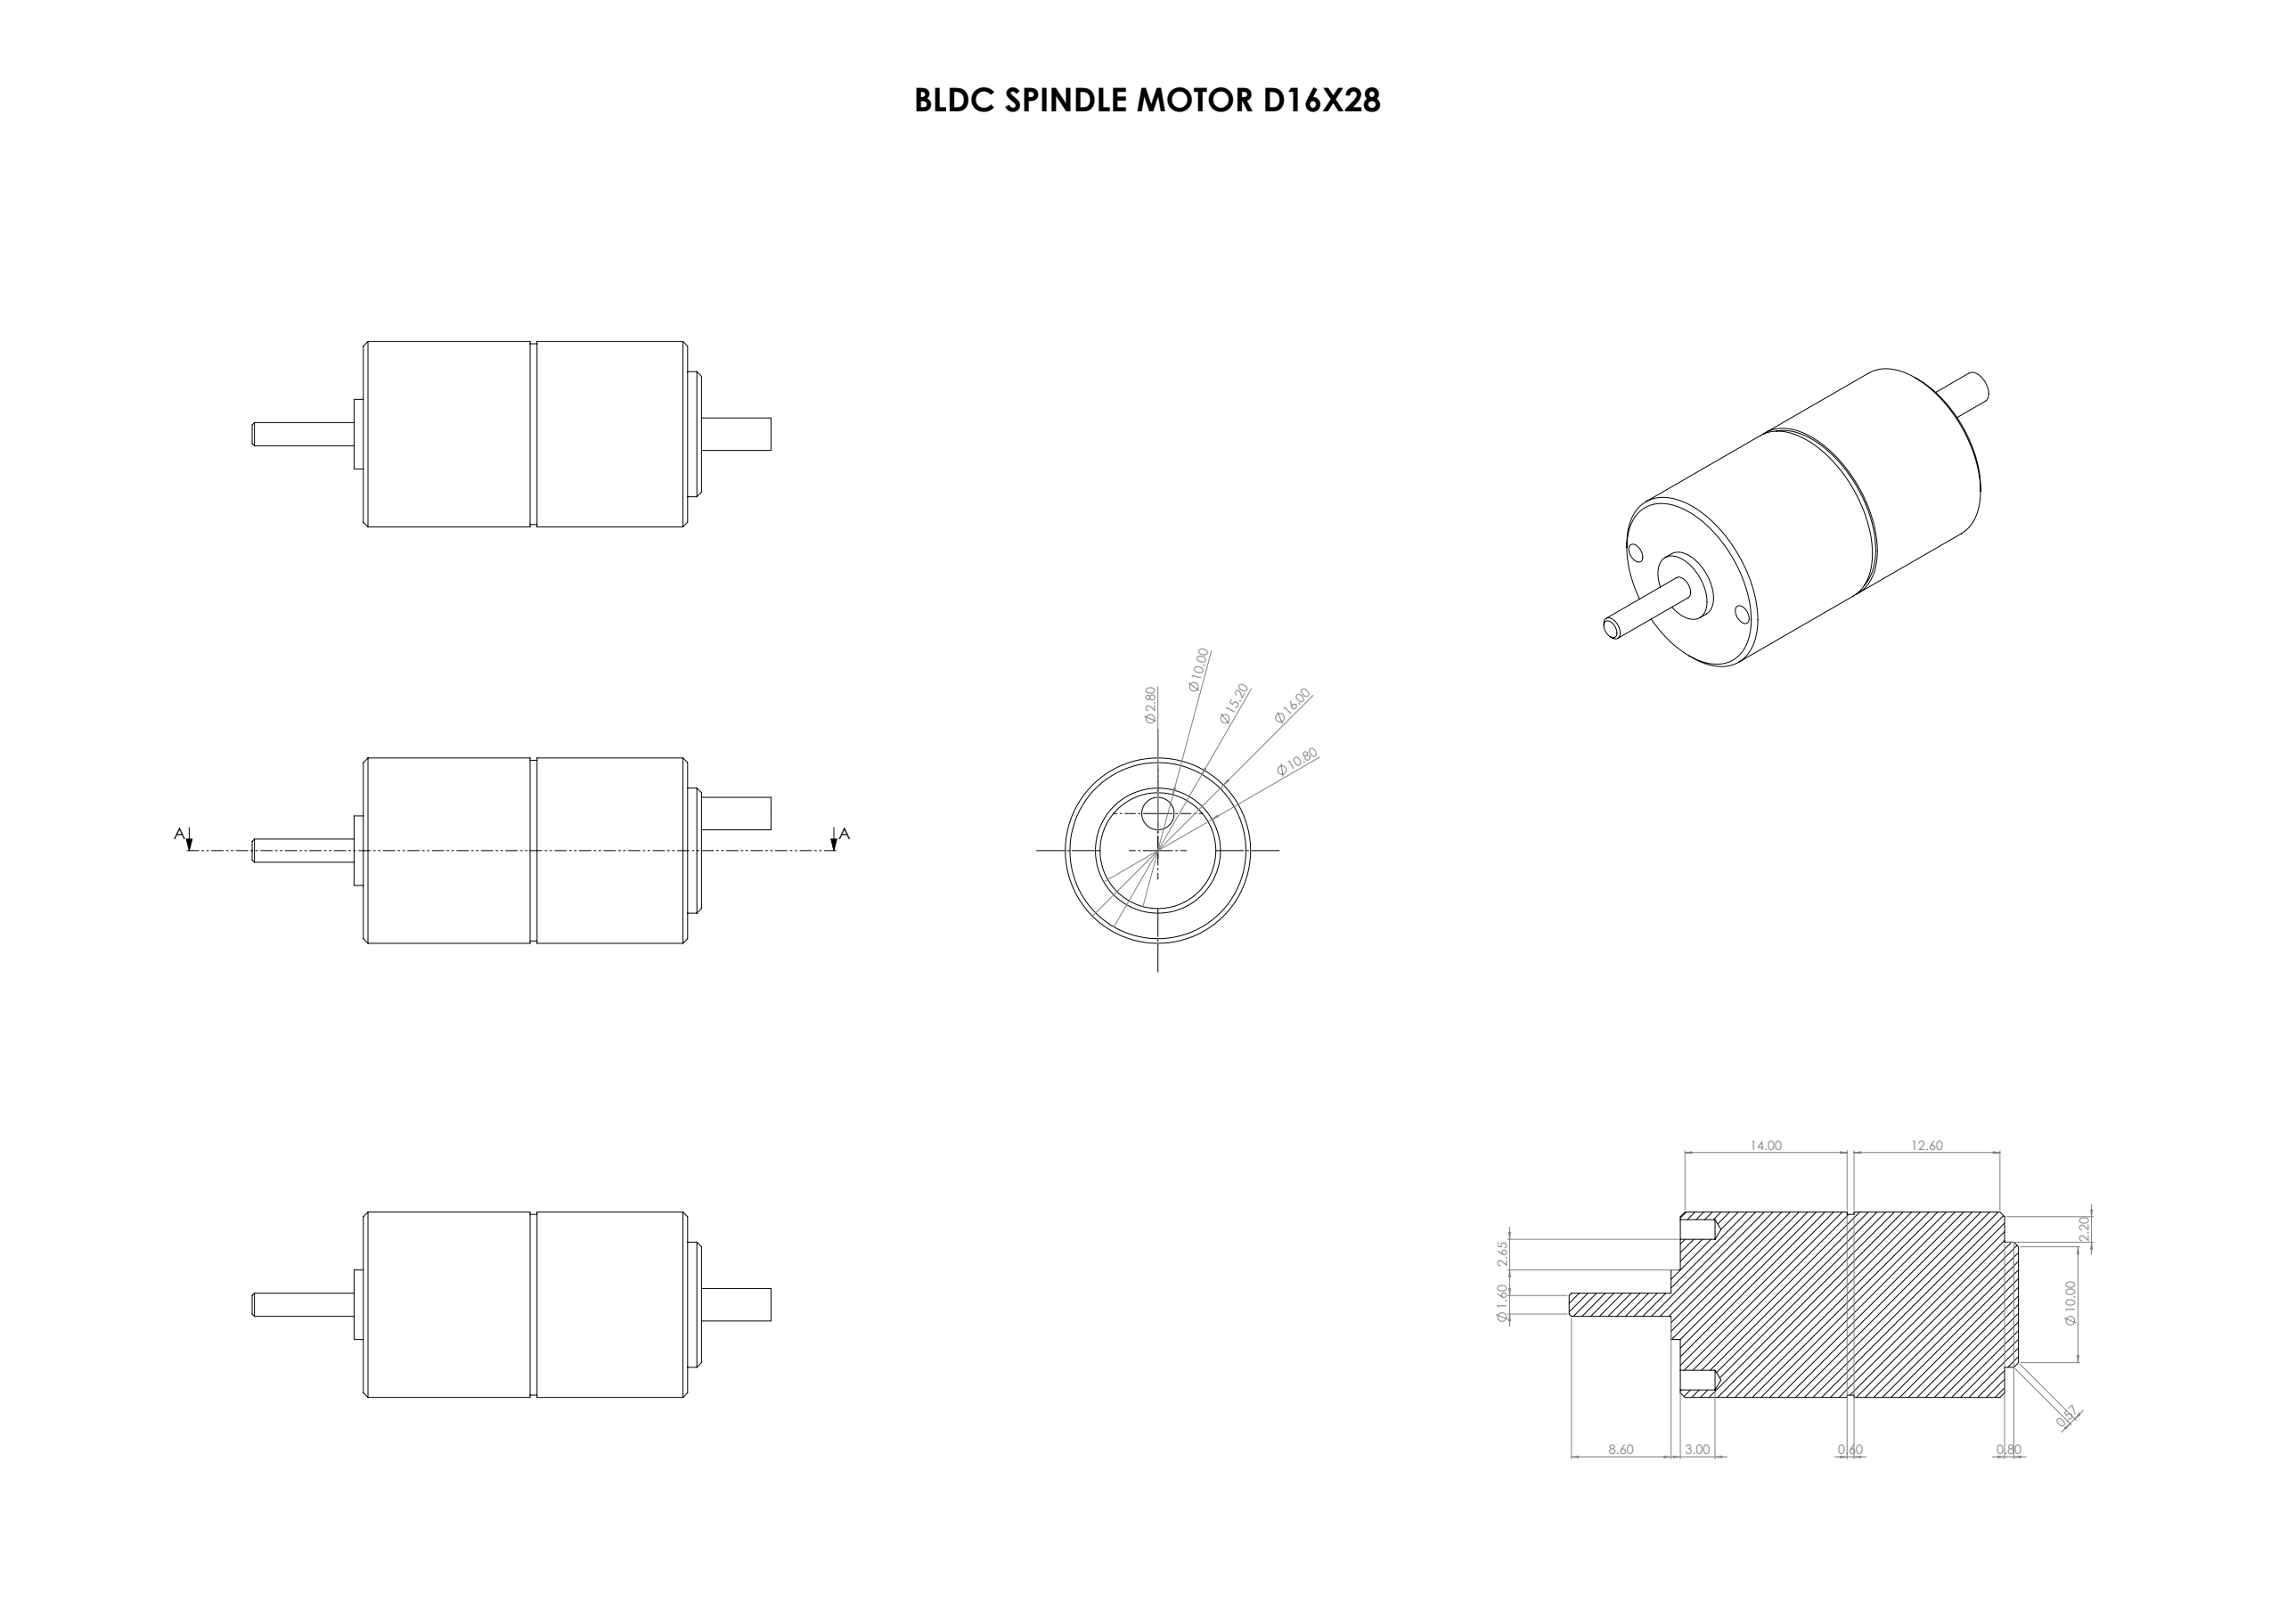
ISO-10303-21;
HEADER;
/* Generated by software containing ST-Developer
 * from STEP Tools, Inc. (www.steptools.com) 
 */

FILE_DESCRIPTION(
/* description */ (''),
/* implementation_level */ '2;1');

FILE_NAME(
/* name */ '07_BLDC_Spindle_Motor_D16x28.step',
/* time_stamp */ '2026-10-19T23:00:43-07:00',
/* author */ (''),
/* organization */ (''),
/* preprocessor_version */ 'ST-DEVELOPER v20.2',
/* originating_system */ 'Autodesk Translation Framework v15.15.0.0',
/* authorisation */ '');

FILE_SCHEMA (('AUTOMOTIVE_DESIGN { 1 0 10303 214 3 1 1 }'));
ENDSEC;

DATA;
#10=MECHANICAL_DESIGN_GEOMETRIC_PRESENTATION_REPRESENTATION('',(#1002),#55002);
#962=SHAPE_REPRESENTATION_RELATIONSHIP('SRR','None',#55110,#982);
#982=ADVANCED_BREP_SHAPE_REPRESENTATION('',(#1022),#54988);
#1002=STYLED_ITEM('',(#55372),#1022);
#1022=MANIFOLD_SOLID_BREP('BLDC Motor',#24535);
#1189=FACE_BOUND('',#4421,.T.);
#1190=FACE_BOUND('',#4426,.T.);
#1191=FACE_BOUND('',#4428,.T.);
#1192=FACE_BOUND('',#4431,.T.);
#1193=FACE_BOUND('',#4436,.T.);
#1194=FACE_BOUND('',#4437,.T.);
#1195=FACE_BOUND('',#4438,.T.);
#1196=FACE_BOUND('',#4441,.T.);
#1425=PLANE('',#25811);
#1426=PLANE('',#25812);
#1427=PLANE('',#25821);
#1428=PLANE('',#25823);
#1429=PLANE('',#25827);
#1430=PLANE('',#25834);
#1431=PLANE('',#25838);
#1432=PLANE('',#25844);
#2139=CYLINDRICAL_SURFACE('',#25802,0.085);
#2140=CYLINDRICAL_SURFACE('',#25806,0.085);
#2141=CYLINDRICAL_SURFACE('',#25808,0.14);
#2142=CYLINDRICAL_SURFACE('',#25816,0.54);
#2143=CYLINDRICAL_SURFACE('',#25818,0.78);
#2144=CYLINDRICAL_SURFACE('',#25825,0.8);
#2145=CYLINDRICAL_SURFACE('',#25831,0.8);
#2146=CYLINDRICAL_SURFACE('',#25836,0.3);
#2147=CYLINDRICAL_SURFACE('',#25840,0.1);
#2897=FACE_OUTER_BOUND('',#4414,.T.);
#2898=FACE_OUTER_BOUND('',#4415,.T.);
#2899=FACE_OUTER_BOUND('',#4416,.T.);
#2900=FACE_OUTER_BOUND('',#4417,.T.);
#2901=FACE_OUTER_BOUND('',#4418,.T.);
#2902=FACE_OUTER_BOUND('',#4419,.T.);
#2903=FACE_OUTER_BOUND('',#4420,.T.);
#2904=FACE_OUTER_BOUND('',#4422,.T.);
#2905=FACE_OUTER_BOUND('',#4423,.T.);
#2906=FACE_OUTER_BOUND('',#4424,.T.);
#2907=FACE_OUTER_BOUND('',#4425,.T.);
#2908=FACE_OUTER_BOUND('',#4427,.T.);
#2909=FACE_OUTER_BOUND('',#4429,.T.);
#2910=FACE_OUTER_BOUND('',#4430,.T.);
#2911=FACE_OUTER_BOUND('',#4432,.T.);
#2912=FACE_OUTER_BOUND('',#4433,.T.);
#2913=FACE_OUTER_BOUND('',#4434,.T.);
#2914=FACE_OUTER_BOUND('',#4435,.T.);
#2915=FACE_OUTER_BOUND('',#4439,.T.);
#2916=FACE_OUTER_BOUND('',#4440,.T.);
#2917=FACE_OUTER_BOUND('',#4442,.T.);
#2918=FACE_OUTER_BOUND('',#4443,.T.);
#2919=FACE_OUTER_BOUND('',#4444,.T.);
#4414=EDGE_LOOP('',(#18100,#18101,#18102));
#4415=EDGE_LOOP('',(#18103,#18104,#18105,#18106));
#4416=EDGE_LOOP('',(#18107,#18108,#18109));
#4417=EDGE_LOOP('',(#18110,#18111,#18112,#18113));
#4418=EDGE_LOOP('',(#18114,#18115,#18116,#18117));
#4419=EDGE_LOOP('',(#18118));
#4420=EDGE_LOOP('',(#18119));
#4421=EDGE_LOOP('',(#18120));
#4422=EDGE_LOOP('',(#18121,#18122,#18123,#18124));
#4423=EDGE_LOOP('',(#18125,#18126,#18127,#18128));
#4424=EDGE_LOOP('',(#18129,#18130,#18131,#18132));
#4425=EDGE_LOOP('',(#18133));
#4426=EDGE_LOOP('',(#18134));
#4427=EDGE_LOOP('',(#18135));
#4428=EDGE_LOOP('',(#18136));
#4429=EDGE_LOOP('',(#18137,#18138,#18139,#18140));
#4430=EDGE_LOOP('',(#18141));
#4431=EDGE_LOOP('',(#18142));
#4432=EDGE_LOOP('',(#18143,#18144,#18145,#18146));
#4433=EDGE_LOOP('',(#18147,#18148,#18149,#18150));
#4434=EDGE_LOOP('',(#18151,#18152,#18153,#18154));
#4435=EDGE_LOOP('',(#18155));
#4436=EDGE_LOOP('',(#18156));
#4437=EDGE_LOOP('',(#18157));
#4438=EDGE_LOOP('',(#18158));
#4439=EDGE_LOOP('',(#18159,#18160,#18161,#18162));
#4440=EDGE_LOOP('',(#18163));
#4441=EDGE_LOOP('',(#18164));
#4442=EDGE_LOOP('',(#18165,#18166,#18167,#18168));
#4443=EDGE_LOOP('',(#18169,#18170,#18171,#18172));
#4444=EDGE_LOOP('',(#18173));
#5948=LINE('',#36207,#7769);
#5949=LINE('',#36211,#7770);
#5950=LINE('',#36216,#7771);
#5951=LINE('',#36220,#7772);
#5952=LINE('',#36226,#7773);
#5953=LINE('',#36235,#7774);
#5954=LINE('',#36239,#7775);
#5955=LINE('',#36244,#7776);
#5956=LINE('',#36255,#7777);
#5957=LINE('',#36262,#7778);
#5958=LINE('',#36264,#7779);
#5959=LINE('',#36268,#7780);
#5960=LINE('',#36275,#7781);
#5961=LINE('',#36282,#7782);
#5962=LINE('',#36286,#7783);
#7769=VECTOR('',#29826,0.0425);
#7770=VECTOR('',#29831,0.085);
#7771=VECTOR('',#29836,0.0425);
#7772=VECTOR('',#29841,0.085);
#7773=VECTOR('',#29848,0.14);
#7774=VECTOR('',#29861,0.52);
#7775=VECTOR('',#29866,0.54);
#7776=VECTOR('',#29871,0.78);
#7777=VECTOR('',#29886,0.8);
#7778=VECTOR('',#29895,0.78);
#7779=VECTOR('',#29898,0.8);
#7780=VECTOR('',#29903,0.78);
#7781=VECTOR('',#29912,0.3);
#7782=VECTOR('',#29921,0.1);
#7783=VECTOR('',#29926,0.09);
#9559=CIRCLE('',#25801,0.085);
#9560=CIRCLE('',#25803,0.085);
#9561=CIRCLE('',#25805,0.085);
#9562=CIRCLE('',#25807,0.085);
#9563=CIRCLE('',#25809,0.14);
#9564=CIRCLE('',#25810,0.14);
#9565=CIRCLE('',#25813,0.5);
#9566=CIRCLE('',#25815,0.54);
#9567=CIRCLE('',#25817,0.54);
#9568=CIRCLE('',#25819,0.78);
#9569=CIRCLE('',#25820,0.78);
#9570=CIRCLE('',#25822,0.8);
#9571=CIRCLE('',#25824,0.8);
#9572=CIRCLE('',#25826,0.8);
#9573=CIRCLE('',#25828,0.76);
#9574=CIRCLE('',#25830,0.8);
#9575=CIRCLE('',#25833,0.76);
#9576=CIRCLE('',#25835,0.3);
#9577=CIRCLE('',#25837,0.3);
#9578=CIRCLE('',#25839,0.1);
#9579=CIRCLE('',#25841,0.1);
#9580=CIRCLE('',#25843,0.08);
#10743=VERTEX_POINT('',#36205);
#10744=VERTEX_POINT('',#36206);
#10745=VERTEX_POINT('',#36210);
#10746=VERTEX_POINT('',#36214);
#10747=VERTEX_POINT('',#36215);
#10748=VERTEX_POINT('',#36219);
#10749=VERTEX_POINT('',#36223);
#10750=VERTEX_POINT('',#36225);
#10751=VERTEX_POINT('',#36230);
#10752=VERTEX_POINT('',#36233);
#10753=VERTEX_POINT('',#36237);
#10754=VERTEX_POINT('',#36241);
#10755=VERTEX_POINT('',#36243);
#10756=VERTEX_POINT('',#36247);
#10757=VERTEX_POINT('',#36250);
#10758=VERTEX_POINT('',#36253);
#10759=VERTEX_POINT('',#36257);
#10760=VERTEX_POINT('',#36260);
#10761=VERTEX_POINT('',#36266);
#10762=VERTEX_POINT('',#36270);
#10763=VERTEX_POINT('',#36273);
#10764=VERTEX_POINT('',#36277);
#10765=VERTEX_POINT('',#36280);
#10766=VERTEX_POINT('',#36284);
#13458=EDGE_CURVE('',#10743,#10744,#5948,.T.);
#13459=EDGE_CURVE('',#10744,#10744,#9559,.T.);
#13460=EDGE_CURVE('',#10744,#10745,#5949,.T.);
#13461=EDGE_CURVE('',#10745,#10745,#9560,.T.);
#13462=EDGE_CURVE('',#10746,#10747,#5950,.T.);
#13463=EDGE_CURVE('',#10747,#10747,#9561,.T.);
#13464=EDGE_CURVE('',#10747,#10748,#5951,.T.);
#13465=EDGE_CURVE('',#10748,#10748,#9562,.T.);
#13466=EDGE_CURVE('',#10749,#10749,#9563,.T.);
#13467=EDGE_CURVE('',#10749,#10750,#5952,.T.);
#13468=EDGE_CURVE('',#10750,#10750,#9564,.T.);
#13469=EDGE_CURVE('',#10751,#10751,#9565,.T.);
#13470=EDGE_CURVE('',#10752,#10752,#9566,.T.);
#13471=EDGE_CURVE('',#10752,#10751,#5953,.T.);
#13472=EDGE_CURVE('',#10753,#10753,#9567,.T.);
#13473=EDGE_CURVE('',#10753,#10752,#5954,.T.);
#13474=EDGE_CURVE('',#10754,#10754,#9568,.T.);
#13475=EDGE_CURVE('',#10754,#10755,#5955,.T.);
#13476=EDGE_CURVE('',#10755,#10755,#9569,.T.);
#13477=EDGE_CURVE('',#10756,#10756,#9570,.T.);
#13478=EDGE_CURVE('',#10757,#10757,#9571,.T.);
#13479=EDGE_CURVE('',#10758,#10758,#9572,.T.);
#13480=EDGE_CURVE('',#10758,#10757,#5956,.T.);
#13481=EDGE_CURVE('',#10759,#10759,#9573,.T.);
#13482=EDGE_CURVE('',#10760,#10760,#9574,.T.);
#13483=EDGE_CURVE('',#10760,#10759,#5957,.T.);
#13484=EDGE_CURVE('',#10756,#10760,#5958,.T.);
#13485=EDGE_CURVE('',#10761,#10761,#9575,.T.);
#13486=EDGE_CURVE('',#10761,#10758,#5959,.T.);
#13487=EDGE_CURVE('',#10762,#10762,#9576,.T.);
#13488=EDGE_CURVE('',#10763,#10763,#9577,.T.);
#13489=EDGE_CURVE('',#10763,#10762,#5960,.T.);
#13490=EDGE_CURVE('',#10764,#10764,#9578,.T.);
#13491=EDGE_CURVE('',#10765,#10765,#9579,.T.);
#13492=EDGE_CURVE('',#10765,#10764,#5961,.T.);
#13493=EDGE_CURVE('',#10766,#10766,#9580,.T.);
#13494=EDGE_CURVE('',#10766,#10765,#5962,.T.);
#18100=ORIENTED_EDGE('',*,*,#13458,.T.);
#18101=ORIENTED_EDGE('',*,*,#13459,.T.);
#18102=ORIENTED_EDGE('',*,*,#13458,.F.);
#18103=ORIENTED_EDGE('',*,*,#13459,.F.);
#18104=ORIENTED_EDGE('',*,*,#13460,.T.);
#18105=ORIENTED_EDGE('',*,*,#13461,.F.);
#18106=ORIENTED_EDGE('',*,*,#13460,.F.);
#18107=ORIENTED_EDGE('',*,*,#13462,.T.);
#18108=ORIENTED_EDGE('',*,*,#13463,.T.);
#18109=ORIENTED_EDGE('',*,*,#13462,.F.);
#18110=ORIENTED_EDGE('',*,*,#13463,.F.);
#18111=ORIENTED_EDGE('',*,*,#13464,.T.);
#18112=ORIENTED_EDGE('',*,*,#13465,.F.);
#18113=ORIENTED_EDGE('',*,*,#13464,.F.);
#18114=ORIENTED_EDGE('',*,*,#13466,.F.);
#18115=ORIENTED_EDGE('',*,*,#13467,.T.);
#18116=ORIENTED_EDGE('',*,*,#13468,.F.);
#18117=ORIENTED_EDGE('',*,*,#13467,.F.);
#18118=ORIENTED_EDGE('',*,*,#13466,.T.);
#18119=ORIENTED_EDGE('',*,*,#13469,.F.);
#18120=ORIENTED_EDGE('',*,*,#13468,.T.);
#18121=ORIENTED_EDGE('',*,*,#13470,.F.);
#18122=ORIENTED_EDGE('',*,*,#13471,.T.);
#18123=ORIENTED_EDGE('',*,*,#13469,.T.);
#18124=ORIENTED_EDGE('',*,*,#13471,.F.);
#18125=ORIENTED_EDGE('',*,*,#13472,.F.);
#18126=ORIENTED_EDGE('',*,*,#13473,.T.);
#18127=ORIENTED_EDGE('',*,*,#13470,.T.);
#18128=ORIENTED_EDGE('',*,*,#13473,.F.);
#18129=ORIENTED_EDGE('',*,*,#13474,.T.);
#18130=ORIENTED_EDGE('',*,*,#13475,.T.);
#18131=ORIENTED_EDGE('',*,*,#13476,.F.);
#18132=ORIENTED_EDGE('',*,*,#13475,.F.);
#18133=ORIENTED_EDGE('',*,*,#13477,.F.);
#18134=ORIENTED_EDGE('',*,*,#13474,.F.);
#18135=ORIENTED_EDGE('',*,*,#13478,.F.);
#18136=ORIENTED_EDGE('',*,*,#13476,.T.);
#18137=ORIENTED_EDGE('',*,*,#13479,.F.);
#18138=ORIENTED_EDGE('',*,*,#13480,.T.);
#18139=ORIENTED_EDGE('',*,*,#13478,.T.);
#18140=ORIENTED_EDGE('',*,*,#13480,.F.);
#18141=ORIENTED_EDGE('',*,*,#13481,.F.);
#18142=ORIENTED_EDGE('',*,*,#13472,.T.);
#18143=ORIENTED_EDGE('',*,*,#13482,.F.);
#18144=ORIENTED_EDGE('',*,*,#13483,.T.);
#18145=ORIENTED_EDGE('',*,*,#13481,.T.);
#18146=ORIENTED_EDGE('',*,*,#13483,.F.);
#18147=ORIENTED_EDGE('',*,*,#13477,.T.);
#18148=ORIENTED_EDGE('',*,*,#13484,.T.);
#18149=ORIENTED_EDGE('',*,*,#13482,.T.);
#18150=ORIENTED_EDGE('',*,*,#13484,.F.);
#18151=ORIENTED_EDGE('',*,*,#13485,.F.);
#18152=ORIENTED_EDGE('',*,*,#13486,.T.);
#18153=ORIENTED_EDGE('',*,*,#13479,.T.);
#18154=ORIENTED_EDGE('',*,*,#13486,.F.);
#18155=ORIENTED_EDGE('',*,*,#13485,.T.);
#18156=ORIENTED_EDGE('',*,*,#13461,.T.);
#18157=ORIENTED_EDGE('',*,*,#13465,.T.);
#18158=ORIENTED_EDGE('',*,*,#13487,.F.);
#18159=ORIENTED_EDGE('',*,*,#13488,.F.);
#18160=ORIENTED_EDGE('',*,*,#13489,.T.);
#18161=ORIENTED_EDGE('',*,*,#13487,.T.);
#18162=ORIENTED_EDGE('',*,*,#13489,.F.);
#18163=ORIENTED_EDGE('',*,*,#13488,.T.);
#18164=ORIENTED_EDGE('',*,*,#13490,.F.);
#18165=ORIENTED_EDGE('',*,*,#13491,.F.);
#18166=ORIENTED_EDGE('',*,*,#13492,.T.);
#18167=ORIENTED_EDGE('',*,*,#13490,.T.);
#18168=ORIENTED_EDGE('',*,*,#13492,.F.);
#18169=ORIENTED_EDGE('',*,*,#13493,.F.);
#18170=ORIENTED_EDGE('',*,*,#13494,.T.);
#18171=ORIENTED_EDGE('',*,*,#13491,.T.);
#18172=ORIENTED_EDGE('',*,*,#13494,.F.);
#18173=ORIENTED_EDGE('',*,*,#13493,.T.);
#23103=CONICAL_SURFACE('',#25800,0.0425,1.02974425867665);
#23104=CONICAL_SURFACE('',#25804,0.0425,1.02974425867665);
#23105=CONICAL_SURFACE('',#25814,0.52,0.785398163397448);
#23106=CONICAL_SURFACE('',#25829,0.78,0.785398163397454);
#23107=CONICAL_SURFACE('',#25832,0.78,0.785398163397449);
#23108=CONICAL_SURFACE('',#25842,0.09,0.785398163397451);
#23650=ADVANCED_FACE('',(#2897),#23103,.F.);
#23651=ADVANCED_FACE('',(#2898),#2139,.F.);
#23652=ADVANCED_FACE('',(#2899),#23104,.F.);
#23653=ADVANCED_FACE('',(#2900),#2140,.F.);
#23654=ADVANCED_FACE('',(#2901),#2141,.T.);
#23655=ADVANCED_FACE('',(#2902),#1425,.F.);
#23656=ADVANCED_FACE('',(#2903,#1189),#1426,.T.);
#23657=ADVANCED_FACE('',(#2904),#23105,.T.);
#23658=ADVANCED_FACE('',(#2905),#2142,.T.);
#23659=ADVANCED_FACE('',(#2906),#2143,.T.);
#23660=ADVANCED_FACE('',(#2907,#1190),#1427,.F.);
#23661=ADVANCED_FACE('',(#2908,#1191),#1428,.F.);
#23662=ADVANCED_FACE('',(#2909),#2144,.T.);
#23663=ADVANCED_FACE('',(#2910,#1192),#1429,.T.);
#23664=ADVANCED_FACE('',(#2911),#23106,.T.);
#23665=ADVANCED_FACE('',(#2912),#2145,.T.);
#23666=ADVANCED_FACE('',(#2913),#23107,.T.);
#23667=ADVANCED_FACE('',(#2914,#1193,#1194,#1195),#1430,.T.);
#23668=ADVANCED_FACE('',(#2915),#2146,.T.);
#23669=ADVANCED_FACE('',(#2916,#1196),#1431,.T.);
#23670=ADVANCED_FACE('',(#2917),#2147,.T.);
#23671=ADVANCED_FACE('',(#2918),#23108,.T.);
#23672=ADVANCED_FACE('',(#2919),#1432,.T.);
#24535=CLOSED_SHELL('',(#23650,#23651,#23652,#23653,#23654,#23655,#23656,
#23657,#23658,#23659,#23660,#23661,#23662,#23663,#23664,#23665,#23666,#23667,
#23668,#23669,#23670,#23671,#23672));
#25799=AXIS2_PLACEMENT_3D('',#36203,#29822,#29823);
#25800=AXIS2_PLACEMENT_3D('',#36204,#29824,#29825);
#25801=AXIS2_PLACEMENT_3D('',#36208,#29827,#29828);
#25802=AXIS2_PLACEMENT_3D('',#36209,#29829,#29830);
#25803=AXIS2_PLACEMENT_3D('',#36212,#29832,#29833);
#25804=AXIS2_PLACEMENT_3D('',#36213,#29834,#29835);
#25805=AXIS2_PLACEMENT_3D('',#36217,#29837,#29838);
#25806=AXIS2_PLACEMENT_3D('',#36218,#29839,#29840);
#25807=AXIS2_PLACEMENT_3D('',#36221,#29842,#29843);
#25808=AXIS2_PLACEMENT_3D('',#36222,#29844,#29845);
#25809=AXIS2_PLACEMENT_3D('',#36224,#29846,#29847);
#25810=AXIS2_PLACEMENT_3D('',#36227,#29849,#29850);
#25811=AXIS2_PLACEMENT_3D('',#36228,#29851,#29852);
#25812=AXIS2_PLACEMENT_3D('',#36229,#29853,#29854);
#25813=AXIS2_PLACEMENT_3D('',#36231,#29855,#29856);
#25814=AXIS2_PLACEMENT_3D('',#36232,#29857,#29858);
#25815=AXIS2_PLACEMENT_3D('',#36234,#29859,#29860);
#25816=AXIS2_PLACEMENT_3D('',#36236,#29862,#29863);
#25817=AXIS2_PLACEMENT_3D('',#36238,#29864,#29865);
#25818=AXIS2_PLACEMENT_3D('',#36240,#29867,#29868);
#25819=AXIS2_PLACEMENT_3D('',#36242,#29869,#29870);
#25820=AXIS2_PLACEMENT_3D('',#36245,#29872,#29873);
#25821=AXIS2_PLACEMENT_3D('',#36246,#29874,#29875);
#25822=AXIS2_PLACEMENT_3D('',#36248,#29876,#29877);
#25823=AXIS2_PLACEMENT_3D('',#36249,#29878,#29879);
#25824=AXIS2_PLACEMENT_3D('',#36251,#29880,#29881);
#25825=AXIS2_PLACEMENT_3D('',#36252,#29882,#29883);
#25826=AXIS2_PLACEMENT_3D('',#36254,#29884,#29885);
#25827=AXIS2_PLACEMENT_3D('',#36256,#29887,#29888);
#25828=AXIS2_PLACEMENT_3D('',#36258,#29889,#29890);
#25829=AXIS2_PLACEMENT_3D('',#36259,#29891,#29892);
#25830=AXIS2_PLACEMENT_3D('',#36261,#29893,#29894);
#25831=AXIS2_PLACEMENT_3D('',#36263,#29896,#29897);
#25832=AXIS2_PLACEMENT_3D('',#36265,#29899,#29900);
#25833=AXIS2_PLACEMENT_3D('',#36267,#29901,#29902);
#25834=AXIS2_PLACEMENT_3D('',#36269,#29904,#29905);
#25835=AXIS2_PLACEMENT_3D('',#36271,#29906,#29907);
#25836=AXIS2_PLACEMENT_3D('',#36272,#29908,#29909);
#25837=AXIS2_PLACEMENT_3D('',#36274,#29910,#29911);
#25838=AXIS2_PLACEMENT_3D('',#36276,#29913,#29914);
#25839=AXIS2_PLACEMENT_3D('',#36278,#29915,#29916);
#25840=AXIS2_PLACEMENT_3D('',#36279,#29917,#29918);
#25841=AXIS2_PLACEMENT_3D('',#36281,#29919,#29920);
#25842=AXIS2_PLACEMENT_3D('',#36283,#29922,#29923);
#25843=AXIS2_PLACEMENT_3D('',#36285,#29924,#29925);
#25844=AXIS2_PLACEMENT_3D('',#36287,#29927,#29928);
#29822=DIRECTION('axis',(0.,0.,1.));
#29823=DIRECTION('refdir',(1.,0.,0.));
#29824=DIRECTION('center_axis',(0.,0.,1.));
#29825=DIRECTION('ref_axis',(1.,0.,0.));
#29826=DIRECTION('',(-0.857167300702112,-1.04972719113862E-16,0.515038074910054));
#29827=DIRECTION('center_axis',(0.,0.,1.));
#29828=DIRECTION('ref_axis',(1.,0.,0.));
#29829=DIRECTION('center_axis',(0.,0.,1.));
#29830=DIRECTION('ref_axis',(1.,0.,0.));
#29831=DIRECTION('',(0.,0.,1.));
#29832=DIRECTION('center_axis',(0.,0.,-1.));
#29833=DIRECTION('ref_axis',(1.,0.,0.));
#29834=DIRECTION('center_axis',(0.,0.,1.));
#29835=DIRECTION('ref_axis',(1.,0.,0.));
#29836=DIRECTION('',(-0.857167300702112,-1.04972719113862E-16,0.515038074910054));
#29837=DIRECTION('center_axis',(0.,0.,1.));
#29838=DIRECTION('ref_axis',(1.,0.,0.));
#29839=DIRECTION('center_axis',(0.,0.,1.));
#29840=DIRECTION('ref_axis',(1.,0.,0.));
#29841=DIRECTION('',(0.,0.,1.));
#29842=DIRECTION('center_axis',(0.,0.,-1.));
#29843=DIRECTION('ref_axis',(1.,0.,0.));
#29844=DIRECTION('center_axis',(0.,0.,-1.));
#29845=DIRECTION('ref_axis',(1.,0.,0.));
#29846=DIRECTION('center_axis',(0.,0.,-1.));
#29847=DIRECTION('ref_axis',(1.,0.,0.));
#29848=DIRECTION('',(0.,0.,1.));
#29849=DIRECTION('center_axis',(0.,0.,1.));
#29850=DIRECTION('ref_axis',(1.,0.,0.));
#29851=DIRECTION('center_axis',(0.,0.,1.));
#29852=DIRECTION('ref_axis',(1.,0.,0.));
#29853=DIRECTION('center_axis',(0.,0.,-1.));
#29854=DIRECTION('ref_axis',(-1.,0.,0.));
#29855=DIRECTION('center_axis',(0.,0.,1.));
#29856=DIRECTION('ref_axis',(1.,0.,0.));
#29857=DIRECTION('center_axis',(0.,0.,1.));
#29858=DIRECTION('ref_axis',(1.,0.,0.));
#29859=DIRECTION('center_axis',(0.,0.,1.));
#29860=DIRECTION('ref_axis',(1.,0.,0.));
#29861=DIRECTION('',(0.707106781186548,8.65956056235493E-17,-0.707106781186548));
#29862=DIRECTION('center_axis',(0.,0.,1.));
#29863=DIRECTION('ref_axis',(1.,0.,0.));
#29864=DIRECTION('center_axis',(0.,0.,1.));
#29865=DIRECTION('ref_axis',(1.,0.,0.));
#29866=DIRECTION('',(0.,0.,-1.));
#29867=DIRECTION('center_axis',(0.,0.,1.));
#29868=DIRECTION('ref_axis',(1.,0.,0.));
#29869=DIRECTION('center_axis',(0.,0.,1.));
#29870=DIRECTION('ref_axis',(1.,0.,0.));
#29871=DIRECTION('',(0.,0.,1.));
#29872=DIRECTION('center_axis',(0.,0.,1.));
#29873=DIRECTION('ref_axis',(1.,0.,0.));
#29874=DIRECTION('center_axis',(0.,0.,-1.));
#29875=DIRECTION('ref_axis',(-1.,0.,0.));
#29876=DIRECTION('center_axis',(0.,0.,-1.));
#29877=DIRECTION('ref_axis',(1.,0.,0.));
#29878=DIRECTION('center_axis',(0.,0.,1.));
#29879=DIRECTION('ref_axis',(1.,0.,0.));
#29880=DIRECTION('center_axis',(0.,0.,1.));
#29881=DIRECTION('ref_axis',(1.,0.,0.));
#29882=DIRECTION('center_axis',(0.,0.,1.));
#29883=DIRECTION('ref_axis',(1.,0.,0.));
#29884=DIRECTION('center_axis',(0.,0.,1.));
#29885=DIRECTION('ref_axis',(1.,0.,0.));
#29886=DIRECTION('',(0.,0.,-1.));
#29887=DIRECTION('center_axis',(0.,0.,-1.));
#29888=DIRECTION('ref_axis',(-1.,0.,0.));
#29889=DIRECTION('center_axis',(0.,0.,1.));
#29890=DIRECTION('ref_axis',(1.,0.,0.));
#29891=DIRECTION('center_axis',(0.,0.,1.));
#29892=DIRECTION('ref_axis',(1.,0.,0.));
#29893=DIRECTION('center_axis',(0.,0.,1.));
#29894=DIRECTION('ref_axis',(1.,0.,0.));
#29895=DIRECTION('',(0.707106781186551,8.65956056235498E-17,-0.707106781186544));
#29896=DIRECTION('center_axis',(0.,0.,1.));
#29897=DIRECTION('ref_axis',(1.,0.,0.));
#29898=DIRECTION('',(0.,0.,-1.));
#29899=DIRECTION('center_axis',(0.,0.,-1.));
#29900=DIRECTION('ref_axis',(1.,0.,0.));
#29901=DIRECTION('center_axis',(0.,0.,1.));
#29902=DIRECTION('ref_axis',(1.,0.,0.));
#29903=DIRECTION('',(-0.707106781186548,-8.65956056235494E-17,-0.707106781186547));
#29904=DIRECTION('center_axis',(0.,0.,1.));
#29905=DIRECTION('ref_axis',(1.,0.,0.));
#29906=DIRECTION('center_axis',(0.,0.,1.));
#29907=DIRECTION('ref_axis',(1.,0.,0.));
#29908=DIRECTION('center_axis',(0.,0.,1.));
#29909=DIRECTION('ref_axis',(1.,0.,0.));
#29910=DIRECTION('center_axis',(0.,0.,1.));
#29911=DIRECTION('ref_axis',(1.,0.,0.));
#29912=DIRECTION('',(0.,0.,-1.));
#29913=DIRECTION('center_axis',(0.,0.,1.));
#29914=DIRECTION('ref_axis',(1.,0.,0.));
#29915=DIRECTION('center_axis',(0.,0.,1.));
#29916=DIRECTION('ref_axis',(1.,0.,0.));
#29917=DIRECTION('center_axis',(0.,0.,1.));
#29918=DIRECTION('ref_axis',(1.,0.,0.));
#29919=DIRECTION('center_axis',(0.,0.,1.));
#29920=DIRECTION('ref_axis',(1.,0.,0.));
#29921=DIRECTION('',(0.,0.,-1.));
#29922=DIRECTION('center_axis',(0.,0.,-1.));
#29923=DIRECTION('ref_axis',(1.,0.,0.));
#29924=DIRECTION('center_axis',(0.,0.,1.));
#29925=DIRECTION('ref_axis',(1.,0.,0.));
#29926=DIRECTION('',(-0.707106781186549,-8.65956056235496E-17,-0.707106781186546));
#29927=DIRECTION('center_axis',(0.,0.,1.));
#29928=DIRECTION('ref_axis',(1.,0.,0.));
#36203=CARTESIAN_POINT('',(0.,0.,0.));
#36204=CARTESIAN_POINT('Origin',(-0.65,0.,-0.325536576308671));
#36205=CARTESIAN_POINT('',(-0.65,0.,-0.351073152617343));
#36206=CARTESIAN_POINT('',(-0.735,-1.04094977927525E-17,-0.3));
#36207=CARTESIAN_POINT('',(-0.6925,-5.20474889637625E-18,-0.325536576308671));
#36208=CARTESIAN_POINT('Origin',(-0.65,0.,-0.3));
#36209=CARTESIAN_POINT('Origin',(-0.65,0.,-0.125));
#36210=CARTESIAN_POINT('',(-0.735,1.04094977927525E-17,0.));
#36211=CARTESIAN_POINT('',(-0.735,-1.04094977927525E-17,-0.125));
#36212=CARTESIAN_POINT('Origin',(-0.65,0.,0.));
#36213=CARTESIAN_POINT('Origin',(0.65,0.,-0.325536576308671));
#36214=CARTESIAN_POINT('',(0.65,0.,-0.351073152617343));
#36215=CARTESIAN_POINT('',(0.565,-1.04094977927525E-17,-0.3));
#36216=CARTESIAN_POINT('',(0.6075,-5.20474889637625E-18,-0.325536576308671));
#36217=CARTESIAN_POINT('Origin',(0.65,0.,-0.3));
#36218=CARTESIAN_POINT('Origin',(0.65,0.,-0.125));
#36219=CARTESIAN_POINT('',(0.565,1.04094977927525E-17,0.));
#36220=CARTESIAN_POINT('',(0.565,-1.04094977927525E-17,-0.125));
#36221=CARTESIAN_POINT('Origin',(0.65,0.,0.));
#36222=CARTESIAN_POINT('Origin',(0.,0.32,-2.92));
#36223=CARTESIAN_POINT('',(-0.14,0.32,-3.52));
#36224=CARTESIAN_POINT('Origin',(0.,0.32,-3.52));
#36225=CARTESIAN_POINT('',(-0.14,0.32,-2.92));
#36226=CARTESIAN_POINT('',(-0.14,0.32,-2.92));
#36227=CARTESIAN_POINT('Origin',(0.,0.32,-2.92));
#36228=CARTESIAN_POINT('Origin',(0.,0.32,-3.52));
#36229=CARTESIAN_POINT('Origin',(0.5,0.,-2.92));
#36230=CARTESIAN_POINT('',(-0.5,-6.12323399573677E-17,-2.92));
#36231=CARTESIAN_POINT('Origin',(0.,0.,-2.92));
#36232=CARTESIAN_POINT('Origin',(0.,0.,-2.9));
#36233=CARTESIAN_POINT('',(-0.54,-6.61309271539571E-17,-2.88));
#36234=CARTESIAN_POINT('Origin',(0.,0.,-2.88));
#36235=CARTESIAN_POINT('',(-0.52,-6.36816335556624E-17,-2.9));
#36236=CARTESIAN_POINT('Origin',(0.,0.,-2.84));
#36237=CARTESIAN_POINT('',(-0.54,-6.61309271539571E-17,-2.8));
#36238=CARTESIAN_POINT('Origin',(0.,0.,-2.8));
#36239=CARTESIAN_POINT('',(-0.54,-6.61309271539571E-17,-2.84));
#36240=CARTESIAN_POINT('Origin',(0.,0.,-1.47));
#36241=CARTESIAN_POINT('',(-0.78,-9.55224503334935E-17,-1.5));
#36242=CARTESIAN_POINT('Origin',(0.,0.,-1.5));
#36243=CARTESIAN_POINT('',(-0.78,-9.55224503334935E-17,-1.44));
#36244=CARTESIAN_POINT('',(-0.78,-9.55224503334935E-17,-1.47));
#36245=CARTESIAN_POINT('Origin',(0.,0.,-1.44));
#36246=CARTESIAN_POINT('Origin',(0.82,0.,-1.5));
#36247=CARTESIAN_POINT('',(-0.8,9.79717439317883E-17,-1.5));
#36248=CARTESIAN_POINT('Origin',(0.,0.,-1.5));
#36249=CARTESIAN_POINT('Origin',(0.78,0.,-1.44));
#36250=CARTESIAN_POINT('',(-0.8,-9.79717439317883E-17,-1.44));
#36251=CARTESIAN_POINT('Origin',(0.,0.,-1.44));
#36252=CARTESIAN_POINT('Origin',(0.,0.,-1.4));
#36253=CARTESIAN_POINT('',(-0.8,-9.79717439317883E-17,-0.04));
#36254=CARTESIAN_POINT('Origin',(0.,0.,-0.04));
#36255=CARTESIAN_POINT('',(-0.8,-9.79717439317883E-17,-1.4));
#36256=CARTESIAN_POINT('Origin',(0.76,0.,-2.8));
#36257=CARTESIAN_POINT('',(-0.76,-9.30731567351988E-17,-2.8));
#36258=CARTESIAN_POINT('Origin',(0.,0.,-2.8));
#36259=CARTESIAN_POINT('Origin',(0.,0.,-2.78));
#36260=CARTESIAN_POINT('',(-0.8,-9.79717439317883E-17,-2.76));
#36261=CARTESIAN_POINT('Origin',(0.,0.,-2.76));
#36262=CARTESIAN_POINT('',(-0.78,-9.55224503334935E-17,-2.78));
#36263=CARTESIAN_POINT('Origin',(0.,0.,-1.4));
#36264=CARTESIAN_POINT('',(-0.8,-9.79717439317883E-17,-1.4));
#36265=CARTESIAN_POINT('Origin',(0.,0.,-0.02));
#36266=CARTESIAN_POINT('',(-0.76,-9.30731567351988E-17,-1.04083408558608E-17));
#36267=CARTESIAN_POINT('Origin',(0.,0.,0.));
#36268=CARTESIAN_POINT('',(-0.78,-9.55224503334935E-17,-0.02));
#36269=CARTESIAN_POINT('Origin',(0.3,0.,0.));
#36270=CARTESIAN_POINT('',(-0.3,-3.67394039744206E-17,-6.93889390390723E-18));
#36271=CARTESIAN_POINT('Origin',(0.,0.,0.));
#36272=CARTESIAN_POINT('Origin',(0.,0.,0.04));
#36273=CARTESIAN_POINT('',(-0.3,-3.67394039744206E-17,0.08));
#36274=CARTESIAN_POINT('Origin',(0.,0.,0.08));
#36275=CARTESIAN_POINT('',(-0.3,-3.67394039744206E-17,0.04));
#36276=CARTESIAN_POINT('Origin',(0.1,0.,0.08));
#36277=CARTESIAN_POINT('',(-0.1,-1.22464679914735E-17,0.08));
#36278=CARTESIAN_POINT('Origin',(0.,0.,0.08));
#36279=CARTESIAN_POINT('Origin',(0.,0.,0.51));
#36280=CARTESIAN_POINT('',(-0.1,-1.22464679914735E-17,0.94));
#36281=CARTESIAN_POINT('Origin',(0.,0.,0.94));
#36282=CARTESIAN_POINT('',(-0.1,-1.22464679914735E-17,0.51));
#36283=CARTESIAN_POINT('Origin',(0.,0.,0.95));
#36284=CARTESIAN_POINT('',(-0.08,-9.79717439317882E-18,0.96));
#36285=CARTESIAN_POINT('Origin',(0.,0.,0.96));
#36286=CARTESIAN_POINT('',(-0.09,-1.10218211923262E-17,0.95));
#36287=CARTESIAN_POINT('Origin',(0.,0.,0.96));
#54966=UNCERTAINTY_MEASURE_WITH_UNIT(LENGTH_MEASURE(0.001),#55003,
'DISTANCE_ACCURACY_VALUE',
'Maximum model space distance between geometric entities at asserted c
onnectivities');
#54980=UNCERTAINTY_MEASURE_WITH_UNIT(LENGTH_MEASURE(0.001),#55003,
'DISTANCE_ACCURACY_VALUE',
'Maximum model space distance between geometric entities at asserted c
onnectivities');
#54988=(
GEOMETRIC_REPRESENTATION_CONTEXT(3)
GLOBAL_UNCERTAINTY_ASSIGNED_CONTEXT((#54966))
GLOBAL_UNIT_ASSIGNED_CONTEXT((#55003,#55005,#55006))
REPRESENTATION_CONTEXT('','3D')
);
#55002=(
GEOMETRIC_REPRESENTATION_CONTEXT(3)
GLOBAL_UNCERTAINTY_ASSIGNED_CONTEXT((#54980))
GLOBAL_UNIT_ASSIGNED_CONTEXT((#55003,#55005,#55006))
REPRESENTATION_CONTEXT('','3D')
);
#55003=(
LENGTH_UNIT()
NAMED_UNIT(*)
SI_UNIT(.CENTI.,.METRE.)
);
#55005=(
NAMED_UNIT(*)
PLANE_ANGLE_UNIT()
SI_UNIT($,.RADIAN.)
);
#55006=(
NAMED_UNIT(*)
SI_UNIT($,.STERADIAN.)
SOLID_ANGLE_UNIT()
);
#55014=SHAPE_DEFINITION_REPRESENTATION(#55035,#55110);
#55035=PRODUCT_DEFINITION_SHAPE('',$,#55132);
#55110=SHAPE_REPRESENTATION('',(#25799),#54988);
#55124=PRODUCT_DEFINITION_CONTEXT('part definition',#55189,'design');
#55132=PRODUCT_DEFINITION('2026-10-18-23-36-18-583',
'07_BLDC_Spindle_Motor_D16x28',#55153,#55124);
#55153=PRODUCT_DEFINITION_FORMATION('',$,#55198);
#55189=APPLICATION_CONTEXT(
'Core Data for Automotive Mechanical Design Process');
#55190=PRODUCT_CONTEXT('part definition',#55189,'mechanical');
#55198=PRODUCT('2026-10-18-23-36-18-583','07_BLDC_Spindle_Motor_D16x28',
$,(#55190));
#55366=COLOUR_RGB('Light Blue',0.38,0.62,0.78);
#55367=FILL_AREA_STYLE_COLOUR('',#55366);
#55368=FILL_AREA_STYLE('',(#55367));
#55369=SURFACE_STYLE_FILL_AREA(#55368);
#55370=SURFACE_SIDE_STYLE('',(#55369));
#55371=SURFACE_STYLE_USAGE(.BOTH.,#55370);
#55372=PRESENTATION_STYLE_ASSIGNMENT((#55371));
ENDSEC;
END-ISO-10303-21;
